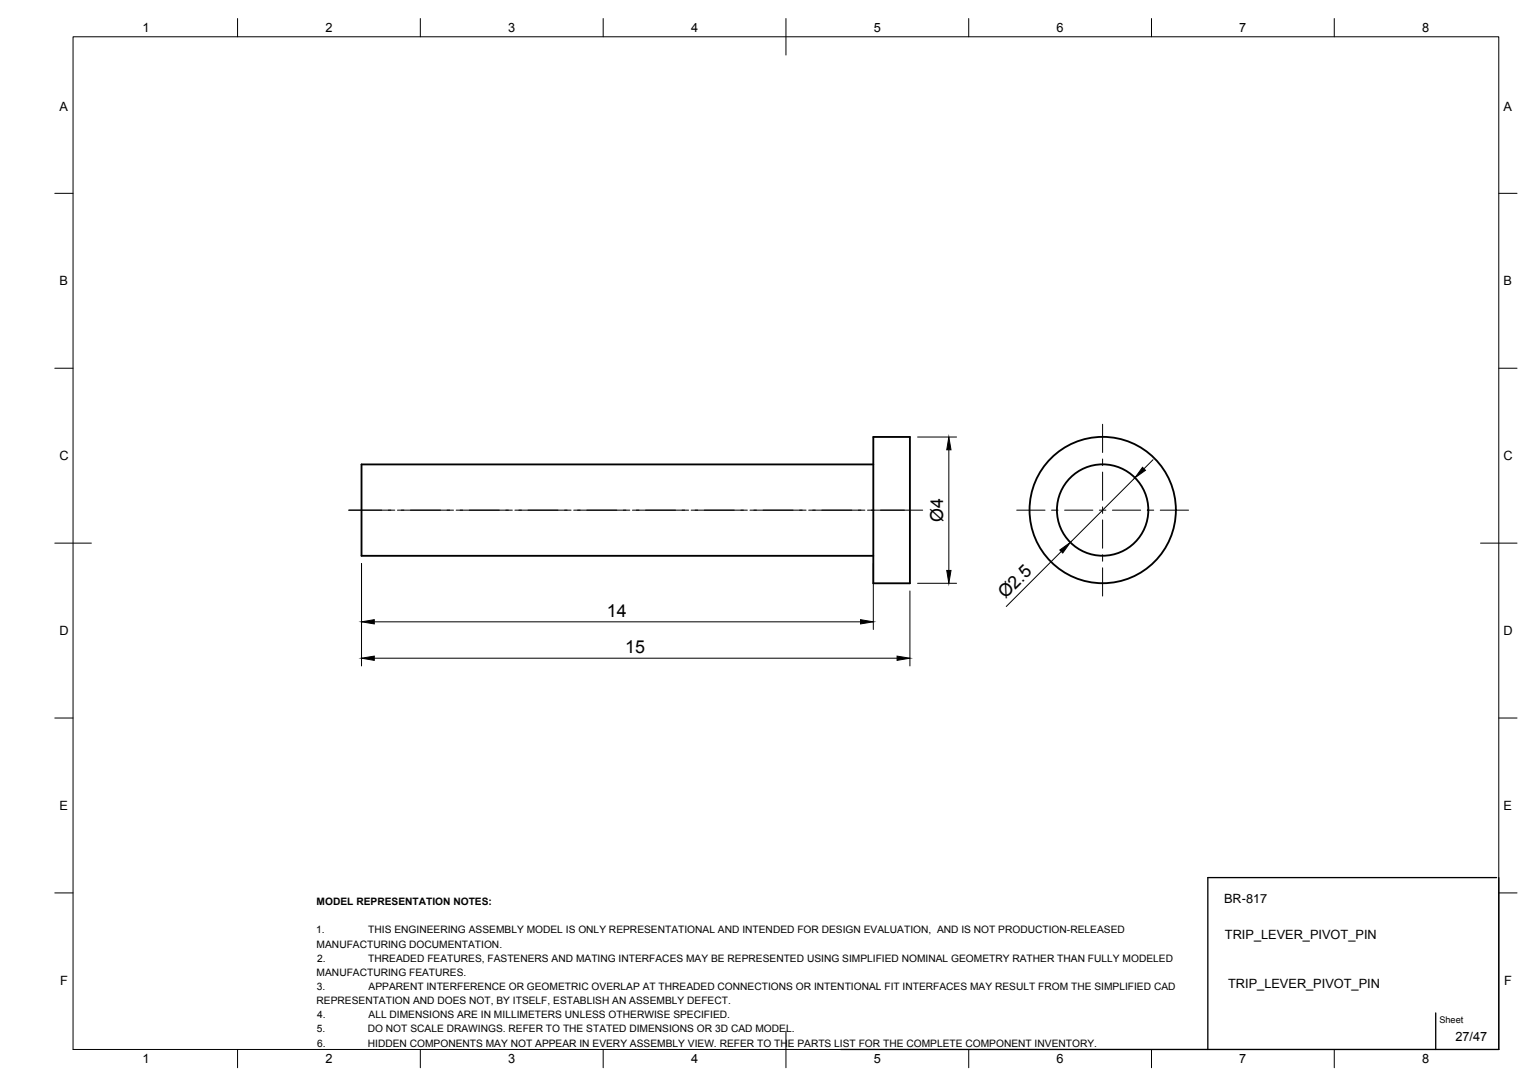
ISO-10303-21;
HEADER;
FILE_DESCRIPTION((''),'2;1');
FILE_NAME('TRIP_LEVER_PIVOT_PIN.step','2026-10-01T22:07:29-07:00',(''),(''),'','','');
FILE_SCHEMA (('AUTOMOTIVE_DESIGN { 1 0 10303 214 3 1 1 }'));
ENDSEC;
DATA;
#10=MECHANICAL_DESIGN_GEOMETRIC_PRESENTATION_REPRESENTATION('',(#559),#15484);
#489=SHAPE_REPRESENTATION_RELATIONSHIP('SRR','None',#15639,#524) ;
#524=ADVANCED_BREP_SHAPE_REPRESENTATION('',(#600),#15463) ;
#559=STYLED_ITEM('',(#15832),#600) ;
#600=MANIFOLD_SOLID_BREP('TRIP_LEVER_PIVOT_PIN',#8270) ;
#686=CYLINDRICAL_SURFACE('',#9038,0.2) ;
#687=CYLINDRICAL_SURFACE('',#9041,0.125) ;
#870=FACE_BOUND('',#2110,.T.) ;
#1015=CIRCLE('',#9036,0.2) ;
#1016=CIRCLE('',#9037,0.125) ;
#1017=CIRCLE('',#9039,0.2) ;
#1018=CIRCLE('',#9042,0.125) ;
#1549=FACE_OUTER_BOUND('',#2109,.T.) ;
#1550=FACE_OUTER_BOUND('',#2111,.T.) ;
#1551=FACE_OUTER_BOUND('',#2112,.T.) ;
#1552=FACE_OUTER_BOUND('',#2113,.T.) ;
#1553=FACE_OUTER_BOUND('',#2114,.T.) ;
#2109=EDGE_LOOP('',(#6015)) ;
#2110=EDGE_LOOP('',(#6016)) ;
#2111=EDGE_LOOP('',(#6017,#6018,#6019,#6020)) ;
#2112=EDGE_LOOP('',(#6021)) ;
#2113=EDGE_LOOP('',(#6022,#6023,#6024,#6025)) ;
#2114=EDGE_LOOP('',(#6026)) ;
#2677=LINE('',#13775,#3151) ;
#2678=LINE('',#13781,#3152) ;
#3151=VECTOR('',#10876,0.2) ;
#3152=VECTOR('',#10885,0.125) ;
#3637=VERTEX_POINT('',#13769) ;
#3638=VERTEX_POINT('',#13771) ;
#3639=VERTEX_POINT('',#13774) ;
#3640=VERTEX_POINT('',#13779) ;
#4512=EDGE_CURVE('',#3637,#3637,#1015,.T.) ;
#4513=EDGE_CURVE('',#3638,#3638,#1016,.T.) ;
#4514=EDGE_CURVE('',#3637,#3639,#2677,.T.) ;
#4515=EDGE_CURVE('',#3639,#3639,#1017,.T.) ;
#4516=EDGE_CURVE('',#3640,#3640,#1018,.T.) ;
#4517=EDGE_CURVE('',#3640,#3638,#2678,.T.) ;
#6015=ORIENTED_EDGE('',*,*,#4512,.T.) ;
#6016=ORIENTED_EDGE('',*,*,#4513,.T.) ;
#6017=ORIENTED_EDGE('',*,*,#4512,.F.) ;
#6018=ORIENTED_EDGE('',*,*,#4514,.T.) ;
#6019=ORIENTED_EDGE('',*,*,#4515,.F.) ;
#6020=ORIENTED_EDGE('',*,*,#4514,.F.) ;
#6021=ORIENTED_EDGE('',*,*,#4515,.T.) ;
#6022=ORIENTED_EDGE('',*,*,#4516,.F.) ;
#6023=ORIENTED_EDGE('',*,*,#4517,.T.) ;
#6024=ORIENTED_EDGE('',*,*,#4513,.F.) ;
#6025=ORIENTED_EDGE('',*,*,#4517,.F.) ;
#6026=ORIENTED_EDGE('',*,*,#4516,.T.) ;
#7655=PLANE('',#9035) ;
#7656=PLANE('',#9040) ;
#7657=PLANE('',#9043) ;
#7936=ADVANCED_FACE('',(#1549,#870),#7655,.T.) ;
#7937=ADVANCED_FACE('',(#1550),#686,.T.) ;
#7938=ADVANCED_FACE('',(#1551),#7656,.T.) ;
#7939=ADVANCED_FACE('',(#1552),#687,.T.) ;
#7940=ADVANCED_FACE('',(#1553),#7657,.T.) ;
#8270=CLOSED_SHELL('',(#7936,#7937,#7938,#7939,#7940)) ;
#9034=AXIS2_PLACEMENT_3D('',#13767,#10866,#10867) ;
#9035=AXIS2_PLACEMENT_3D('',#13768,#10868,#10869) ;
#9036=AXIS2_PLACEMENT_3D('',#13770,#10870,#10871) ;
#9037=AXIS2_PLACEMENT_3D('',#13772,#10872,#10873) ;
#9038=AXIS2_PLACEMENT_3D('',#13773,#10874,#10875) ;
#9039=AXIS2_PLACEMENT_3D('',#13776,#10877,#10878) ;
#9040=AXIS2_PLACEMENT_3D('',#13777,#10879,#10880) ;
#9041=AXIS2_PLACEMENT_3D('',#13778,#10881,#10882) ;
#9042=AXIS2_PLACEMENT_3D('',#13780,#10883,#10884) ;
#9043=AXIS2_PLACEMENT_3D('',#13782,#10886,#10887) ;
#10866=DIRECTION('axis',(0.,0.,1.)) ;
#10867=DIRECTION('refdir',(1.,0.,0.)) ;
#10868=DIRECTION('center_axis',(0.,1.,0.)) ;
#10869=DIRECTION('ref_axis',(1.,0.,0.)) ;
#10870=DIRECTION('center_axis',(0.,1.,0.)) ;
#10871=DIRECTION('ref_axis',(1.,0.,0.)) ;
#10872=DIRECTION('center_axis',(0.,-1.,0.)) ;
#10873=DIRECTION('ref_axis',(1.,0.,0.)) ;
#10874=DIRECTION('center_axis',(0.,1.,0.)) ;
#10875=DIRECTION('ref_axis',(1.,0.,0.)) ;
#10876=DIRECTION('',(0.,-1.,0.)) ;
#10877=DIRECTION('center_axis',(0.,-1.,0.)) ;
#10878=DIRECTION('ref_axis',(1.,0.,0.)) ;
#10879=DIRECTION('center_axis',(0.,-1.,0.)) ;
#10880=DIRECTION('ref_axis',(-1.,0.,0.)) ;
#10881=DIRECTION('center_axis',(0.,1.,0.)) ;
#10882=DIRECTION('ref_axis',(1.,0.,0.)) ;
#10883=DIRECTION('center_axis',(0.,1.,0.)) ;
#10884=DIRECTION('ref_axis',(1.,0.,0.)) ;
#10885=DIRECTION('',(0.,-1.,0.)) ;
#10886=DIRECTION('center_axis',(0.,1.,0.)) ;
#10887=DIRECTION('ref_axis',(1.,0.,0.)) ;
#13767=CARTESIAN_POINT('',(0.,0.,0.)) ;
#13768=CARTESIAN_POINT('Origin',(0.6,0.,2.3)) ;
#13769=CARTESIAN_POINT('',(0.4,0.,2.3)) ;
#13770=CARTESIAN_POINT('Origin',(0.6,0.,2.3)) ;
#13771=CARTESIAN_POINT('',(0.475,0.,2.3)) ;
#13772=CARTESIAN_POINT('Origin',(0.6,0.,2.3)) ;
#13773=CARTESIAN_POINT('Origin',(0.6,-0.05,2.3)) ;
#13774=CARTESIAN_POINT('',(0.4,-0.1,2.3)) ;
#13775=CARTESIAN_POINT('',(0.4,-0.05,2.3)) ;
#13776=CARTESIAN_POINT('Origin',(0.6,-0.1,2.3)) ;
#13777=CARTESIAN_POINT('Origin',(0.6,-0.1,2.3)) ;
#13778=CARTESIAN_POINT('Origin',(0.6,0.7,2.3)) ;
#13779=CARTESIAN_POINT('',(0.475,1.4,2.3)) ;
#13780=CARTESIAN_POINT('Origin',(0.6,1.4,2.3)) ;
#13781=CARTESIAN_POINT('',(0.475,0.7,2.3)) ;
#13782=CARTESIAN_POINT('Origin',(0.6,1.4,2.3)) ;
#15420=UNCERTAINTY_MEASURE_WITH_UNIT(LENGTH_MEASURE(0.001),#15485,
'DISTANCE_ACCURACY_VALUE',
'Maximum model space distance between geometric entities at asserted c
onnectivities') ;
#15441=UNCERTAINTY_MEASURE_WITH_UNIT(LENGTH_MEASURE(0.001),#15485,
'DISTANCE_ACCURACY_VALUE',
'Maximum model space distance between geometric entities at asserted c
onnectivities') ;
#15463=(
GEOMETRIC_REPRESENTATION_CONTEXT(3)
GLOBAL_UNCERTAINTY_ASSIGNED_CONTEXT((#15420))
GLOBAL_UNIT_ASSIGNED_CONTEXT((#15485,#15487,#15488))
REPRESENTATION_CONTEXT('','3D')
) ;
#15484=(
GEOMETRIC_REPRESENTATION_CONTEXT(3)
GLOBAL_UNCERTAINTY_ASSIGNED_CONTEXT((#15441))
GLOBAL_UNIT_ASSIGNED_CONTEXT((#15485,#15487,#15488))
REPRESENTATION_CONTEXT('','3D')
) ;
#15485=(
LENGTH_UNIT()
NAMED_UNIT(*)
SI_UNIT(.CENTI.,.METRE.)
) ;
#15487=(
NAMED_UNIT(*)
PLANE_ANGLE_UNIT()
SI_UNIT($,.RADIAN.)
) ;
#15488=(
NAMED_UNIT(*)
SI_UNIT($,.STERADIAN.)
SOLID_ANGLE_UNIT()
) ;
#15510=SHAPE_DEFINITION_REPRESENTATION(#15567,#15639) ;
#15567=PRODUCT_DEFINITION_SHAPE('',$,#15682) ;
#15639=SHAPE_REPRESENTATION('',(#9034),#15463) ;
#15660=PRODUCT_DEFINITION_CONTEXT('part definition',#15788,'design') ;
#15682=PRODUCT_DEFINITION('TRIP_LEVER_PIVOT_PIN',
'TRIP_LEVER_PIVOT_PIN',#15724,#15660) ;
#15724=PRODUCT_DEFINITION_FORMATION('',$,#15811) ;
#15788=APPLICATION_CONTEXT(
'Core Data for Automotive Mechanical Design Process') ;
#15789=PRODUCT_CONTEXT('part definition',#15788,'mechanical') ;
#15811=PRODUCT('TRIP_LEVER_PIVOT_PIN','TRIP_LEVER_PIVOT_PIN',$,(#15789)) ;
#15832=PRESENTATION_STYLE_ASSIGNMENT((#15844)) ;
#15844=SURFACE_STYLE_USAGE(.BOTH.,#15856) ;
#15856=SURFACE_SIDE_STYLE('',(#15868)) ;
#15868=SURFACE_STYLE_FILL_AREA(#15880) ;
#15880=FILL_AREA_STYLE('Steel - Satin',(#15892)) ;
#15892=FILL_AREA_STYLE_COLOUR('Steel - Satin',#15904) ;
#15904=COLOUR_RGB('Steel - Satin', 0.72549020, 0.75294118, 0.79215686) ;
ENDSEC;
END-ISO-10303-21;
